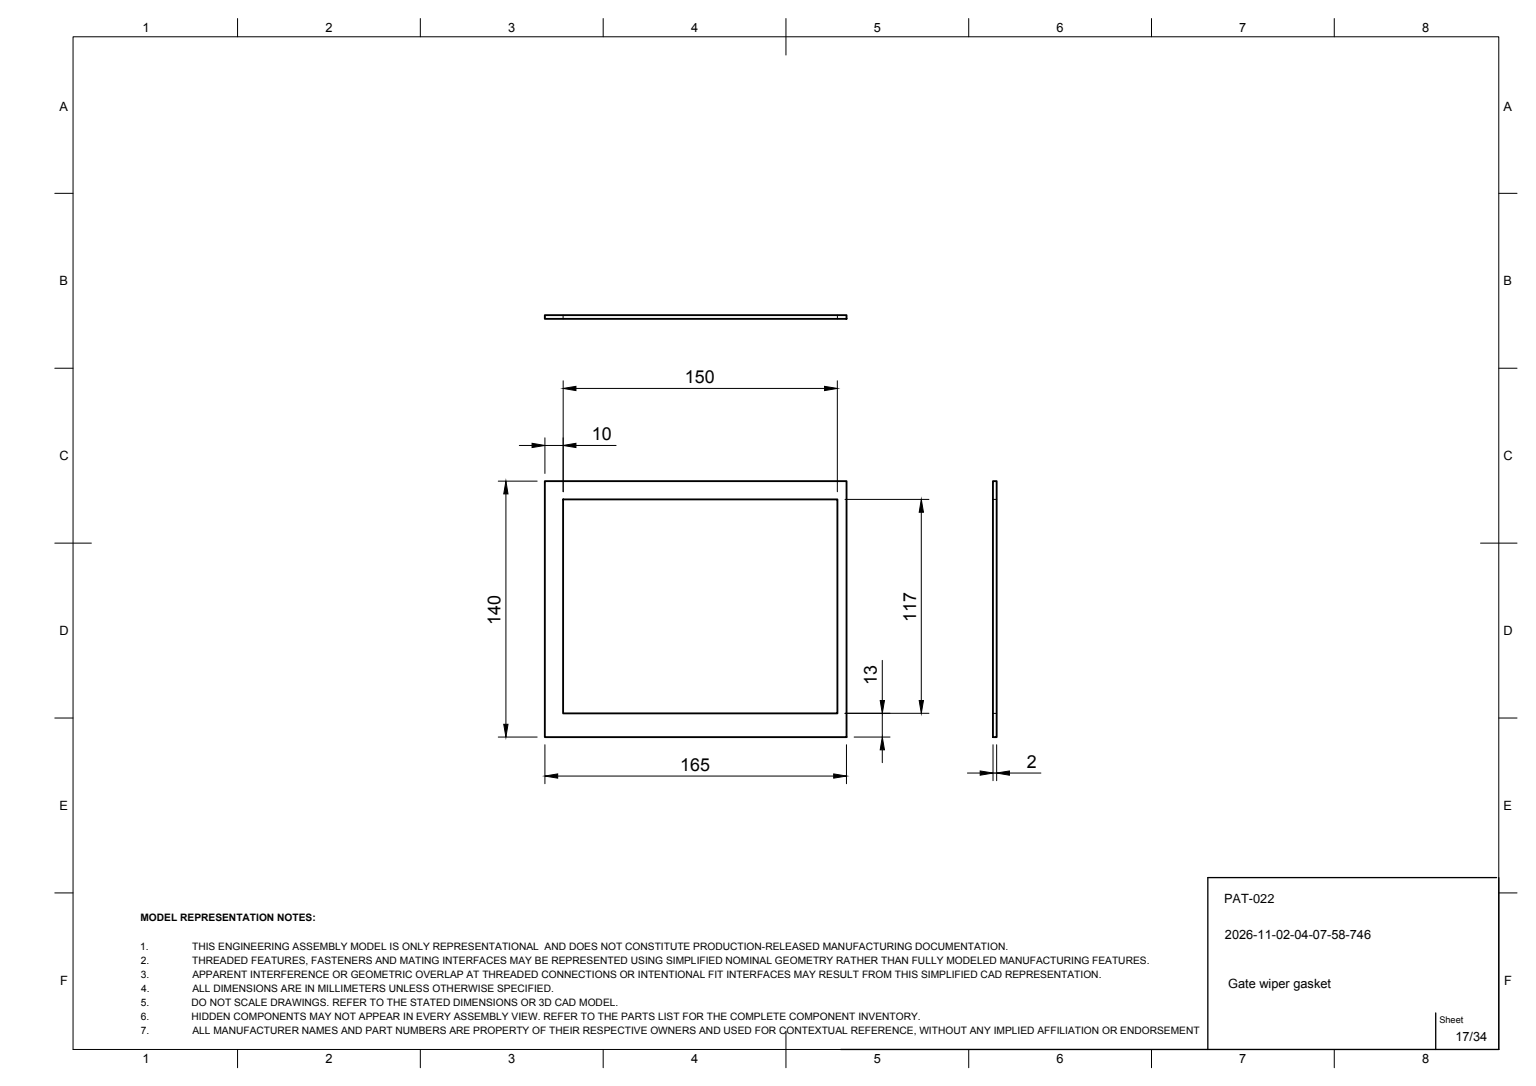
ISO-10303-21;
HEADER;
/* Generated by software containing ST-Developer
 * from STEP Tools, Inc. (www.steptools.com) 
 */

FILE_DESCRIPTION(
/* description */ ('Chute with adjustable gate'),
/* implementation_level */ '2;1');

FILE_NAME(
/* name */ 'Gate wiper gasket.step',
/* time_stamp */ '2026-10-27T10:52:28-07:00',
/* author */ (''),
/* organization */ (''),
/* preprocessor_version */ 'ST-DEVELOPER v20.2',
/* originating_system */ 'Autodesk Translation Framework v15.17.0.0',
/* authorisation */ '');

FILE_SCHEMA (('AUTOMOTIVE_DESIGN { 1 0 10303 214 3 1 1 }'));
ENDSEC;

DATA;
#10=MECHANICAL_DESIGN_GEOMETRIC_PRESENTATION_REPRESENTATION('',(#426),#13094);
#362=SHAPE_REPRESENTATION_RELATIONSHIP('SRR','None',#13263,#394);
#394=ADVANCED_BREP_SHAPE_REPRESENTATION('',(#458),#13072);
#426=STYLED_ITEM('',(#13481),#458);
#458=MANIFOLD_SOLID_BREP('Body1',#7609);
#518=FACE_BOUND('',#1494,.T.);
#519=FACE_BOUND('',#1496,.T.);
#678=PLANE('',#8161);
#679=PLANE('',#8162);
#680=PLANE('',#8163);
#681=PLANE('',#8164);
#682=PLANE('',#8165);
#683=PLANE('',#8166);
#684=PLANE('',#8167);
#685=PLANE('',#8168);
#686=PLANE('',#8169);
#687=PLANE('',#8170);
#1026=FACE_OUTER_BOUND('',#1485,.T.);
#1027=FACE_OUTER_BOUND('',#1486,.T.);
#1028=FACE_OUTER_BOUND('',#1487,.T.);
#1029=FACE_OUTER_BOUND('',#1488,.T.);
#1030=FACE_OUTER_BOUND('',#1489,.T.);
#1031=FACE_OUTER_BOUND('',#1490,.T.);
#1032=FACE_OUTER_BOUND('',#1491,.T.);
#1033=FACE_OUTER_BOUND('',#1492,.T.);
#1034=FACE_OUTER_BOUND('',#1493,.T.);
#1035=FACE_OUTER_BOUND('',#1495,.T.);
#1485=EDGE_LOOP('',(#5666,#5667,#5668,#5669));
#1486=EDGE_LOOP('',(#5670,#5671,#5672,#5673));
#1487=EDGE_LOOP('',(#5674,#5675,#5676,#5677));
#1488=EDGE_LOOP('',(#5678,#5679,#5680,#5681));
#1489=EDGE_LOOP('',(#5682,#5683,#5684,#5685));
#1490=EDGE_LOOP('',(#5686,#5687,#5688,#5689));
#1491=EDGE_LOOP('',(#5690,#5691,#5692,#5693));
#1492=EDGE_LOOP('',(#5694,#5695,#5696,#5697));
#1493=EDGE_LOOP('',(#5698,#5699,#5700,#5701));
#1494=EDGE_LOOP('',(#5702,#5703,#5704,#5705));
#1495=EDGE_LOOP('',(#5706,#5707,#5708,#5709));
#1496=EDGE_LOOP('',(#5710,#5711,#5712,#5713));
#2052=LINE('',#11429,#2829);
#2053=LINE('',#11431,#2830);
#2054=LINE('',#11433,#2831);
#2055=LINE('',#11434,#2832);
#2056=LINE('',#11437,#2833);
#2057=LINE('',#11439,#2834);
#2058=LINE('',#11440,#2835);
#2059=LINE('',#11443,#2836);
#2060=LINE('',#11445,#2837);
#2061=LINE('',#11446,#2838);
#2062=LINE('',#11448,#2839);
#2063=LINE('',#11449,#2840);
#2064=LINE('',#11453,#2841);
#2065=LINE('',#11455,#2842);
#2066=LINE('',#11457,#2843);
#2067=LINE('',#11458,#2844);
#2068=LINE('',#11461,#2845);
#2069=LINE('',#11463,#2846);
#2070=LINE('',#11464,#2847);
#2071=LINE('',#11467,#2848);
#2072=LINE('',#11469,#2849);
#2073=LINE('',#11470,#2850);
#2074=LINE('',#11472,#2851);
#2075=LINE('',#11473,#2852);
#2829=VECTOR('',#9242,1.);
#2830=VECTOR('',#9243,1.);
#2831=VECTOR('',#9244,1.);
#2832=VECTOR('',#9245,1.);
#2833=VECTOR('',#9248,1.);
#2834=VECTOR('',#9249,1.);
#2835=VECTOR('',#9250,1.);
#2836=VECTOR('',#9253,1.);
#2837=VECTOR('',#9254,1.);
#2838=VECTOR('',#9255,1.);
#2839=VECTOR('',#9258,1.);
#2840=VECTOR('',#9259,1.);
#2841=VECTOR('',#9262,1.);
#2842=VECTOR('',#9263,1.);
#2843=VECTOR('',#9264,1.);
#2844=VECTOR('',#9265,1.);
#2845=VECTOR('',#9268,1.);
#2846=VECTOR('',#9269,1.);
#2847=VECTOR('',#9270,1.);
#2848=VECTOR('',#9273,1.);
#2849=VECTOR('',#9274,1.);
#2850=VECTOR('',#9275,1.);
#2851=VECTOR('',#9278,1.);
#2852=VECTOR('',#9279,1.);
#3753=VERTEX_POINT('',#11427);
#3754=VERTEX_POINT('',#11428);
#3755=VERTEX_POINT('',#11430);
#3756=VERTEX_POINT('',#11432);
#3757=VERTEX_POINT('',#11436);
#3758=VERTEX_POINT('',#11438);
#3759=VERTEX_POINT('',#11442);
#3760=VERTEX_POINT('',#11444);
#3761=VERTEX_POINT('',#11451);
#3762=VERTEX_POINT('',#11452);
#3763=VERTEX_POINT('',#11454);
#3764=VERTEX_POINT('',#11456);
#3765=VERTEX_POINT('',#11460);
#3766=VERTEX_POINT('',#11462);
#3767=VERTEX_POINT('',#11466);
#3768=VERTEX_POINT('',#11468);
#4466=EDGE_CURVE('',#3753,#3754,#2052,.T.);
#4467=EDGE_CURVE('',#3755,#3753,#2053,.T.);
#4468=EDGE_CURVE('',#3756,#3755,#2054,.T.);
#4469=EDGE_CURVE('',#3756,#3754,#2055,.T.);
#4470=EDGE_CURVE('',#3754,#3757,#2056,.T.);
#4471=EDGE_CURVE('',#3758,#3756,#2057,.T.);
#4472=EDGE_CURVE('',#3758,#3757,#2058,.T.);
#4473=EDGE_CURVE('',#3757,#3759,#2059,.T.);
#4474=EDGE_CURVE('',#3760,#3758,#2060,.T.);
#4475=EDGE_CURVE('',#3760,#3759,#2061,.T.);
#4476=EDGE_CURVE('',#3759,#3753,#2062,.T.);
#4477=EDGE_CURVE('',#3755,#3760,#2063,.T.);
#4478=EDGE_CURVE('',#3761,#3762,#2064,.T.);
#4479=EDGE_CURVE('',#3762,#3763,#2065,.T.);
#4480=EDGE_CURVE('',#3764,#3763,#2066,.T.);
#4481=EDGE_CURVE('',#3761,#3764,#2067,.T.);
#4482=EDGE_CURVE('',#3765,#3761,#2068,.T.);
#4483=EDGE_CURVE('',#3766,#3764,#2069,.T.);
#4484=EDGE_CURVE('',#3765,#3766,#2070,.T.);
#4485=EDGE_CURVE('',#3767,#3765,#2071,.T.);
#4486=EDGE_CURVE('',#3768,#3766,#2072,.T.);
#4487=EDGE_CURVE('',#3767,#3768,#2073,.T.);
#4488=EDGE_CURVE('',#3762,#3767,#2074,.T.);
#4489=EDGE_CURVE('',#3763,#3768,#2075,.T.);
#5666=ORIENTED_EDGE('',*,*,#4466,.F.);
#5667=ORIENTED_EDGE('',*,*,#4467,.F.);
#5668=ORIENTED_EDGE('',*,*,#4468,.F.);
#5669=ORIENTED_EDGE('',*,*,#4469,.T.);
#5670=ORIENTED_EDGE('',*,*,#4470,.F.);
#5671=ORIENTED_EDGE('',*,*,#4469,.F.);
#5672=ORIENTED_EDGE('',*,*,#4471,.F.);
#5673=ORIENTED_EDGE('',*,*,#4472,.T.);
#5674=ORIENTED_EDGE('',*,*,#4473,.F.);
#5675=ORIENTED_EDGE('',*,*,#4472,.F.);
#5676=ORIENTED_EDGE('',*,*,#4474,.F.);
#5677=ORIENTED_EDGE('',*,*,#4475,.T.);
#5678=ORIENTED_EDGE('',*,*,#4476,.F.);
#5679=ORIENTED_EDGE('',*,*,#4475,.F.);
#5680=ORIENTED_EDGE('',*,*,#4477,.F.);
#5681=ORIENTED_EDGE('',*,*,#4467,.T.);
#5682=ORIENTED_EDGE('',*,*,#4478,.T.);
#5683=ORIENTED_EDGE('',*,*,#4479,.T.);
#5684=ORIENTED_EDGE('',*,*,#4480,.F.);
#5685=ORIENTED_EDGE('',*,*,#4481,.F.);
#5686=ORIENTED_EDGE('',*,*,#4482,.T.);
#5687=ORIENTED_EDGE('',*,*,#4481,.T.);
#5688=ORIENTED_EDGE('',*,*,#4483,.F.);
#5689=ORIENTED_EDGE('',*,*,#4484,.F.);
#5690=ORIENTED_EDGE('',*,*,#4485,.T.);
#5691=ORIENTED_EDGE('',*,*,#4484,.T.);
#5692=ORIENTED_EDGE('',*,*,#4486,.F.);
#5693=ORIENTED_EDGE('',*,*,#4487,.F.);
#5694=ORIENTED_EDGE('',*,*,#4488,.T.);
#5695=ORIENTED_EDGE('',*,*,#4487,.T.);
#5696=ORIENTED_EDGE('',*,*,#4489,.F.);
#5697=ORIENTED_EDGE('',*,*,#4479,.F.);
#5698=ORIENTED_EDGE('',*,*,#4489,.T.);
#5699=ORIENTED_EDGE('',*,*,#4486,.T.);
#5700=ORIENTED_EDGE('',*,*,#4483,.T.);
#5701=ORIENTED_EDGE('',*,*,#4480,.T.);
#5702=ORIENTED_EDGE('',*,*,#4473,.T.);
#5703=ORIENTED_EDGE('',*,*,#4476,.T.);
#5704=ORIENTED_EDGE('',*,*,#4466,.T.);
#5705=ORIENTED_EDGE('',*,*,#4470,.T.);
#5706=ORIENTED_EDGE('',*,*,#4488,.F.);
#5707=ORIENTED_EDGE('',*,*,#4478,.F.);
#5708=ORIENTED_EDGE('',*,*,#4482,.F.);
#5709=ORIENTED_EDGE('',*,*,#4485,.F.);
#5710=ORIENTED_EDGE('',*,*,#4474,.T.);
#5711=ORIENTED_EDGE('',*,*,#4471,.T.);
#5712=ORIENTED_EDGE('',*,*,#4468,.T.);
#5713=ORIENTED_EDGE('',*,*,#4477,.T.);
#7294=ADVANCED_FACE('',(#1026),#678,.F.);
#7295=ADVANCED_FACE('',(#1027),#679,.F.);
#7296=ADVANCED_FACE('',(#1028),#680,.F.);
#7297=ADVANCED_FACE('',(#1029),#681,.F.);
#7298=ADVANCED_FACE('',(#1030),#682,.T.);
#7299=ADVANCED_FACE('',(#1031),#683,.T.);
#7300=ADVANCED_FACE('',(#1032),#684,.T.);
#7301=ADVANCED_FACE('',(#1033),#685,.T.);
#7302=ADVANCED_FACE('',(#1034,#518),#686,.T.);
#7303=ADVANCED_FACE('',(#1035,#519),#687,.F.);
#7609=CLOSED_SHELL('',(#7294,#7295,#7296,#7297,#7298,#7299,#7300,#7301,
#7302,#7303));
#8160=AXIS2_PLACEMENT_3D('',#11425,#9238,#9239);
#8161=AXIS2_PLACEMENT_3D('',#11426,#9240,#9241);
#8162=AXIS2_PLACEMENT_3D('',#11435,#9246,#9247);
#8163=AXIS2_PLACEMENT_3D('',#11441,#9251,#9252);
#8164=AXIS2_PLACEMENT_3D('',#11447,#9256,#9257);
#8165=AXIS2_PLACEMENT_3D('',#11450,#9260,#9261);
#8166=AXIS2_PLACEMENT_3D('',#11459,#9266,#9267);
#8167=AXIS2_PLACEMENT_3D('',#11465,#9271,#9272);
#8168=AXIS2_PLACEMENT_3D('',#11471,#9276,#9277);
#8169=AXIS2_PLACEMENT_3D('',#11474,#9280,#9281);
#8170=AXIS2_PLACEMENT_3D('',#11475,#9282,#9283);
#9238=DIRECTION('axis',(0.,0.,1.));
#9239=DIRECTION('refdir',(1.,0.,0.));
#9240=DIRECTION('center_axis',(0.,0.,-1.));
#9241=DIRECTION('ref_axis',(0.,1.,0.));
#9242=DIRECTION('',(0.,-1.,0.));
#9243=DIRECTION('',(1.,0.,0.));
#9244=DIRECTION('',(0.,1.,0.));
#9245=DIRECTION('',(1.,0.,0.));
#9246=DIRECTION('center_axis',(0.,-1.,0.));
#9247=DIRECTION('ref_axis',(0.,0.,-1.));
#9248=DIRECTION('',(0.,0.,1.));
#9249=DIRECTION('',(0.,0.,-1.));
#9250=DIRECTION('',(1.,0.,0.));
#9251=DIRECTION('center_axis',(0.,0.,1.));
#9252=DIRECTION('ref_axis',(0.,-1.,0.));
#9253=DIRECTION('',(0.,1.,0.));
#9254=DIRECTION('',(0.,-1.,0.));
#9255=DIRECTION('',(1.,0.,0.));
#9256=DIRECTION('center_axis',(0.,1.,0.));
#9257=DIRECTION('ref_axis',(0.,0.,1.));
#9258=DIRECTION('',(0.,0.,-1.));
#9259=DIRECTION('',(0.,0.,1.));
#9260=DIRECTION('center_axis',(0.,0.,1.));
#9261=DIRECTION('ref_axis',(0.,-1.,0.));
#9262=DIRECTION('',(0.,-1.,0.));
#9263=DIRECTION('',(1.,0.,0.));
#9264=DIRECTION('',(0.,-1.,0.));
#9265=DIRECTION('',(1.,0.,0.));
#9266=DIRECTION('center_axis',(0.,1.,0.));
#9267=DIRECTION('ref_axis',(0.,0.,1.));
#9268=DIRECTION('',(0.,0.,1.));
#9269=DIRECTION('',(0.,0.,1.));
#9270=DIRECTION('',(1.,0.,0.));
#9271=DIRECTION('center_axis',(0.,0.,-1.));
#9272=DIRECTION('ref_axis',(0.,1.,0.));
#9273=DIRECTION('',(0.,1.,0.));
#9274=DIRECTION('',(0.,1.,0.));
#9275=DIRECTION('',(1.,0.,0.));
#9276=DIRECTION('center_axis',(0.,-1.,0.));
#9277=DIRECTION('ref_axis',(0.,0.,-1.));
#9278=DIRECTION('',(0.,0.,-1.));
#9279=DIRECTION('',(0.,0.,-1.));
#9280=DIRECTION('center_axis',(1.,0.,0.));
#9281=DIRECTION('ref_axis',(0.,0.,-1.));
#9282=DIRECTION('center_axis',(1.,0.,0.));
#9283=DIRECTION('ref_axis',(0.,0.,-1.));
#11425=CARTESIAN_POINT('',(0.,0.,0.));
#11426=CARTESIAN_POINT('Origin',(-1.3,-7.5,4.3));
#11427=CARTESIAN_POINT('',(-1.,7.5,4.3));
#11428=CARTESIAN_POINT('',(-1.,-7.5,4.3));
#11429=CARTESIAN_POINT('',(-1.,-3.625,4.3));
#11430=CARTESIAN_POINT('',(-1.2,7.5,4.3));
#11431=CARTESIAN_POINT('',(-1.3,7.5,4.3));
#11432=CARTESIAN_POINT('',(-1.2,-7.5,4.3));
#11433=CARTESIAN_POINT('',(-1.2,-3.625,4.3));
#11434=CARTESIAN_POINT('',(-1.3,-7.5,4.3));
#11435=CARTESIAN_POINT('Origin',(-1.3,-7.5,16.));
#11436=CARTESIAN_POINT('',(-1.,-7.5,16.));
#11437=CARTESIAN_POINT('',(-1.,-7.5,13.));
#11438=CARTESIAN_POINT('',(-1.2,-7.5,16.));
#11439=CARTESIAN_POINT('',(-1.2,-7.5,13.));
#11440=CARTESIAN_POINT('',(-1.3,-7.5,16.));
#11441=CARTESIAN_POINT('Origin',(-1.3,7.5,16.));
#11442=CARTESIAN_POINT('',(-1.,7.5,16.));
#11443=CARTESIAN_POINT('',(-1.,3.875,16.));
#11444=CARTESIAN_POINT('',(-1.2,7.5,16.));
#11445=CARTESIAN_POINT('',(-1.2,3.875,16.));
#11446=CARTESIAN_POINT('',(-1.3,7.5,16.));
#11447=CARTESIAN_POINT('Origin',(-1.3,7.5,4.3));
#11448=CARTESIAN_POINT('',(-1.,7.5,7.15));
#11449=CARTESIAN_POINT('',(-1.2,7.5,7.15));
#11450=CARTESIAN_POINT('Origin',(-1.2,8.5,17.));
#11451=CARTESIAN_POINT('',(-1.2,8.5,17.));
#11452=CARTESIAN_POINT('',(-1.2,-8.,17.));
#11453=CARTESIAN_POINT('',(-1.2,8.5,17.));
#11454=CARTESIAN_POINT('',(-1.,-8.,17.));
#11455=CARTESIAN_POINT('',(-1.2,-8.,17.));
#11456=CARTESIAN_POINT('',(-1.,8.5,17.));
#11457=CARTESIAN_POINT('',(-1.,8.5,17.));
#11458=CARTESIAN_POINT('',(-1.2,8.5,17.));
#11459=CARTESIAN_POINT('Origin',(-1.2,8.5,3.));
#11460=CARTESIAN_POINT('',(-1.2,8.5,3.));
#11461=CARTESIAN_POINT('',(-1.2,8.5,3.));
#11462=CARTESIAN_POINT('',(-1.,8.5,3.));
#11463=CARTESIAN_POINT('',(-1.,8.5,3.));
#11464=CARTESIAN_POINT('',(-1.2,8.5,3.));
#11465=CARTESIAN_POINT('Origin',(-1.2,-8.,3.));
#11466=CARTESIAN_POINT('',(-1.2,-8.,3.));
#11467=CARTESIAN_POINT('',(-1.2,-8.,3.));
#11468=CARTESIAN_POINT('',(-1.,-8.,3.));
#11469=CARTESIAN_POINT('',(-1.,-8.,3.));
#11470=CARTESIAN_POINT('',(-1.2,-8.,3.));
#11471=CARTESIAN_POINT('Origin',(-1.2,-8.,17.));
#11472=CARTESIAN_POINT('',(-1.2,-8.,17.));
#11473=CARTESIAN_POINT('',(-1.,-8.,17.));
#11474=CARTESIAN_POINT('Origin',(-1.,0.25,10.));
#11475=CARTESIAN_POINT('Origin',(-1.2,0.25,10.));
#13035=UNCERTAINTY_MEASURE_WITH_UNIT(LENGTH_MEASURE(0.001),#13095,
'DISTANCE_ACCURACY_VALUE',
'Maximum model space distance between geometric entities at asserted c
onnectivities');
#13057=UNCERTAINTY_MEASURE_WITH_UNIT(LENGTH_MEASURE(0.001),#13095,
'DISTANCE_ACCURACY_VALUE',
'Maximum model space distance between geometric entities at asserted c
onnectivities');
#13072=(
GEOMETRIC_REPRESENTATION_CONTEXT(3)
GLOBAL_UNCERTAINTY_ASSIGNED_CONTEXT((#13035))
GLOBAL_UNIT_ASSIGNED_CONTEXT((#13095,#13097,#13098))
REPRESENTATION_CONTEXT('','3D')
);
#13094=(
GEOMETRIC_REPRESENTATION_CONTEXT(3)
GLOBAL_UNCERTAINTY_ASSIGNED_CONTEXT((#13057))
GLOBAL_UNIT_ASSIGNED_CONTEXT((#13095,#13097,#13098))
REPRESENTATION_CONTEXT('','3D')
);
#13095=(
LENGTH_UNIT()
NAMED_UNIT(*)
SI_UNIT(.CENTI.,.METRE.)
);
#13097=(
NAMED_UNIT(*)
PLANE_ANGLE_UNIT()
SI_UNIT($,.RADIAN.)
);
#13098=(
NAMED_UNIT(*)
SI_UNIT($,.STERADIAN.)
SOLID_ANGLE_UNIT()
);
#13113=SHAPE_DEFINITION_REPRESENTATION(#13149,#13263);
#13149=PRODUCT_DEFINITION_SHAPE('',$,#13300);
#13263=SHAPE_REPRESENTATION('',(#8160),#13072);
#13285=PRODUCT_DEFINITION_CONTEXT('part definition',#13395,'design');
#13300=PRODUCT_DEFINITION('Gate wiper gasket','Gate wiper gasket',#13336,
#13285);
#13336=PRODUCT_DEFINITION_FORMATION('',$,#13411);
#13395=APPLICATION_CONTEXT(
'Core Data for Automotive Mechanical Design Process');
#13396=PRODUCT_CONTEXT('part definition',#13395,'mechanical');
#13411=PRODUCT('Gate wiper gasket','Gate wiper gasket',
'Gate wiper gasket',(#13396));
#13475=COLOUR_RGB('Light Blue',0.38,0.62,0.78);
#13476=FILL_AREA_STYLE_COLOUR('',#13475);
#13477=FILL_AREA_STYLE('',(#13476));
#13478=SURFACE_STYLE_FILL_AREA(#13477);
#13479=SURFACE_SIDE_STYLE('',(#13478));
#13480=SURFACE_STYLE_USAGE(.BOTH.,#13479);
#13481=PRESENTATION_STYLE_ASSIGNMENT((#13480));
ENDSEC;
END-ISO-10303-21;
